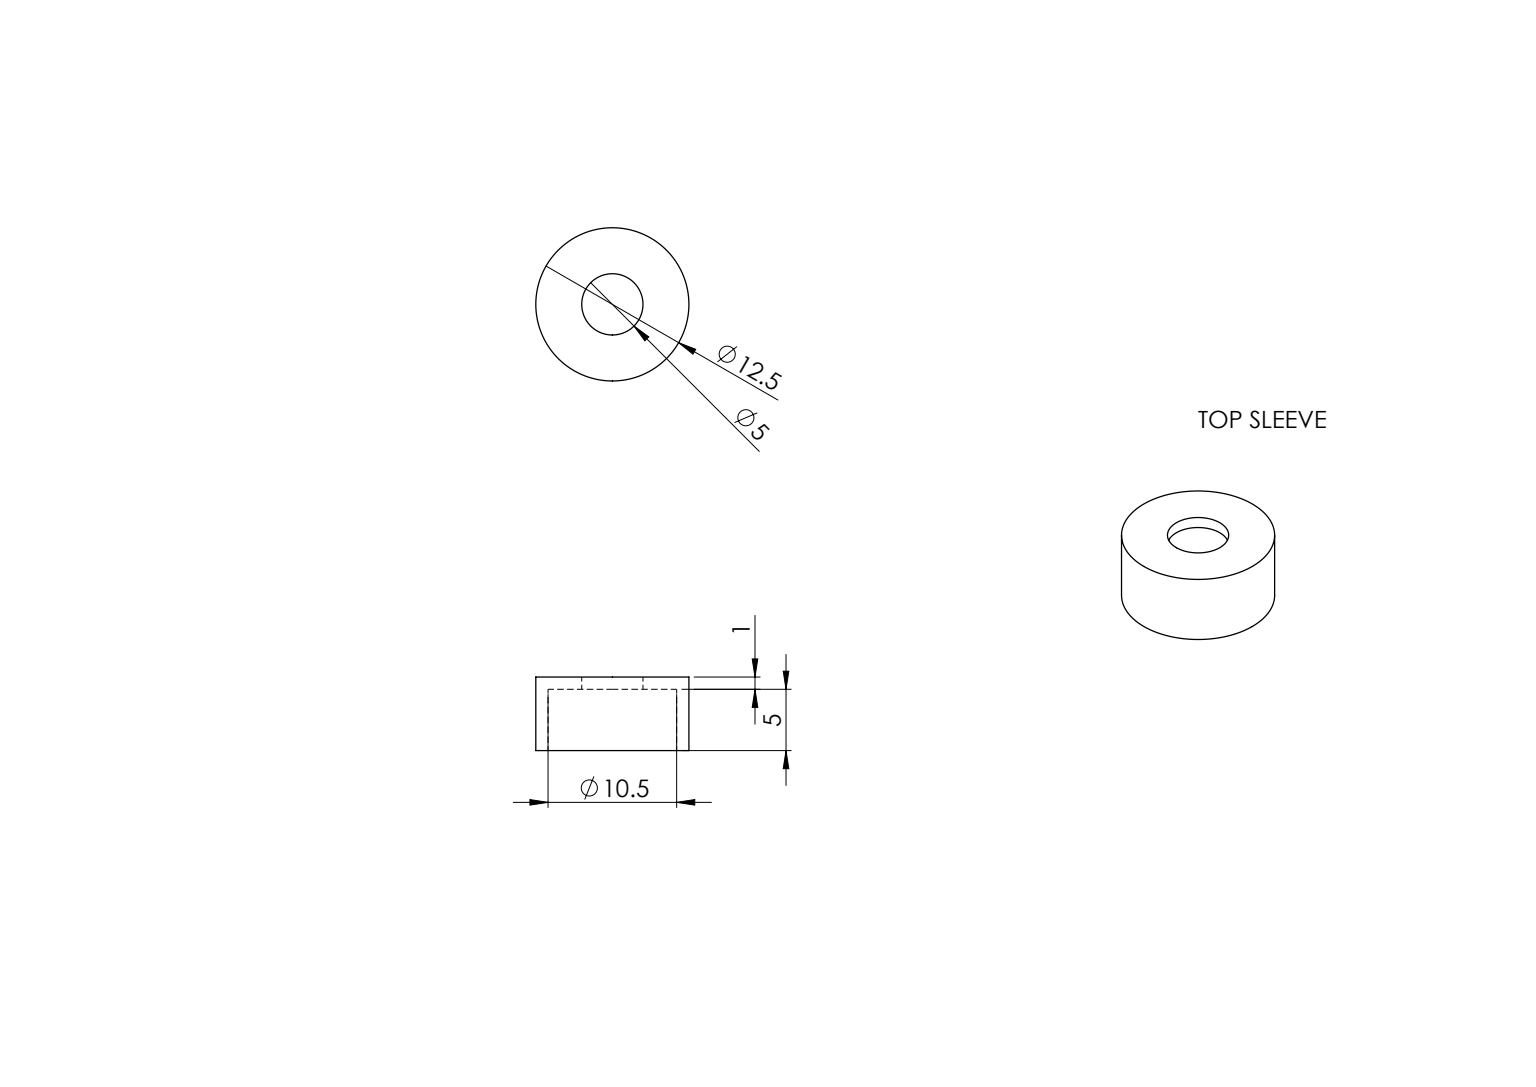
ISO-10303-21;
HEADER;
FILE_DESCRIPTION (('STEP AP214'),
    '1' );
FILE_NAME ('top sleeve.step',
    '2026-10-27T10:49:47',
    ( '' ),
    ( '' ),
    'SwSTEP 2.0',
    'SolidWorks 2026',
    '' );
FILE_SCHEMA (( 'AUTOMOTIVE_DESIGN' ));
ENDSEC;

DATA;
#1=ORIENTED_EDGE ( 'NONE', *, *, #5722, .T. ) ;
#2=FILL_AREA_STYLE ('',( #5004 ) ) ;
#66=EDGE_LOOP ( 'NONE', ( #5126, #5183, #1901, #2100 ) ) ;
#73=CYLINDRICAL_SURFACE ( 'NONE', #5825, 2.499999999999999556 ) ;
#128=DIRECTION ( 'NONE',  ( 0.000000000000000000, 0.000000000000000000, 1.000000000000000000 ) ) ;
#129=AXIS2_PLACEMENT_3D ( 'NONE', #454, #8273, #5425 ) ;
#179=VERTEX_POINT ( 'NONE', #5659 ) ;
#187=VERTEX_POINT ( 'NONE', #5479 ) ;
#213=DIRECTION ( 'NONE',  ( 0.000000000000000000, 1.000000000000000000, 0.000000000000000000 ) ) ;
#302=AXIS2_PLACEMENT_3D ( 'NONE', #4792, #7636, #6980 ) ;
#320=ORIENTED_EDGE ( 'NONE', *, *, #3522, .T. ) ;
#446=STYLED_ITEM('',(#9211),#2174);
#454=CARTESIAN_POINT ( 'NONE',  ( 0.000000000000000000, 69.99999999999998579, 0.000000000000000000 ) ) ;
#543=CARTESIAN_POINT ( 'NONE',  ( 0.000000000000000000, 69.99999999999998579, 0.000000000000000000 ) ) ;
#587=FACE_BOUND ( 'NONE', #2803, .T. ) ;
#600=AXIS2_PLACEMENT_3D ( 'NONE', #1254, #6968, #5476 ) ;
#654=( LENGTH_UNIT ( ) NAMED_UNIT ( * ) SI_UNIT ( .MILLI., .METRE. ) );
#666=CARTESIAN_POINT ( 'NONE',  ( 0.000000000000000000, 76.00000000000000000, -2.499999999999999556 ) ) ;
#689=CARTESIAN_POINT ( 'NONE',  ( 3.061616997868382648E-16, 76.00000000000000000, 2.499999999999999556 ) ) ;
#693=( NAMED_UNIT ( * ) PLANE_ANGLE_UNIT ( ) SI_UNIT ( $, .RADIAN. ) );
#736=ORIENTED_EDGE ( 'NONE', *, *, #3059, .T. ) ;
#780=AXIS2_PLACEMENT_3D ( 'NONE', #6952, #8529, #7794 ) ;
#805=DIRECTION ( 'NONE',  ( 0.000000000000000000, 1.000000000000000000, 0.000000000000000000 ) ) ;
#808=EDGE_LOOP ( 'NONE', ( #7978, #931, #7565, #1484 ) ) ;
#827=CARTESIAN_POINT ( 'NONE',  ( 0.000000000000000000, 75.00000000000000000, 0.000000000000000000 ) ) ;
#850=MECHANICAL_DESIGN_GEOMETRIC_PRESENTATION_REPRESENTATION('',(#4576),#5468);
#856=ORIENTED_EDGE ( 'NONE', *, *, #3685, .T. ) ;
#888=AXIS2_PLACEMENT_3D ( 'NONE', #4026, #9081, #6861 ) ;
#890=CIRCLE ( 'NONE', #3281, 5.250000000000000000 ) ;
#909=CARTESIAN_POINT ( 'NONE',  ( 0.000000000000000000, 75.00000000000000000, 0.000000000000000000 ) ) ;
#931=ORIENTED_EDGE ( 'NONE', *, *, #6120, .T. ) ;
#957=EDGE_CURVE ( 'NONE', #7496, #1130, #5197, .T. ) ;
#992=ORIENTED_EDGE ( 'NONE', *, *, #8749, .T. ) ;
#1009=PRODUCT_DEFINITION_FORMATION_WITH_SPECIFIED_SOURCE ( 'ANY', '', #1433, .NOT_KNOWN. ) ;
#1032=DIRECTION ( 'NONE',  ( 0.000000000000000000, 0.000000000000000000, 1.000000000000000000 ) ) ;
#1088=FACE_OUTER_BOUND ( 'NONE', #5599, .T. ) ;
#1125=EDGE_CURVE ( 'NONE', #8145, #1171, #1682, .T. ) ;
#1130=VERTEX_POINT ( 'NONE', #4733 ) ;
#1150=ORIENTED_EDGE ( 'NONE', *, *, #2707, .F. ) ;
#1166=VERTEX_POINT ( 'NONE', #3351 ) ;
#1171=VERTEX_POINT ( 'NONE', #9055 ) ;
#1199=ADVANCED_FACE ( 'NONE', ( #5698 ), #73, .F. ) ;
#1207=AXIS2_PLACEMENT_3D ( 'NONE', #827, #8513, #128 ) ;
#1232=CARTESIAN_POINT ( 'NONE',  ( 0.000000000000000000, 69.99999999999998579, 0.000000000000000000 ) ) ;
#1254=CARTESIAN_POINT ( 'NONE',  ( 0.000000000000000000, 76.00000000000000000, 0.000000000000000000 ) ) ;
#1264=FACE_OUTER_BOUND ( 'NONE', #5853, .T. ) ;
#1380=CARTESIAN_POINT ( 'NONE',  ( 0.000000000000000000, 76.00000000000000000, 0.000000000000000000 ) ) ;
#1396=SURFACE_SIDE_STYLE ('',( #4281 ) ) ;
#1433=PRODUCT ( 'top sleeve', 'top sleeve', '', ( #6229 ) ) ;
#1478=CIRCLE ( 'NONE', #6676, 5.250000000000000000 ) ;
#1484=ORIENTED_EDGE ( 'NONE', *, *, #1125, .F. ) ;
#1487=AXIS2_PLACEMENT_3D ( 'NONE', #3149, #8300, #8894 ) ;
#1496=EDGE_CURVE ( 'NONE', #1166, #179, #8185, .T. ) ;
#1537=DIRECTION ( 'NONE',  ( 0.000000000000000000, 1.000000000000000000, 0.000000000000000000 ) ) ;
#1623=ORIENTED_EDGE ( 'NONE', *, *, #8749, .F. ) ;
#1627=EDGE_LOOP ( 'NONE', ( #6721, #320, #992, #4948 ) ) ;
#1682=CIRCLE ( 'NONE', #6140, 6.250000000000000000 ) ;
#1693=CIRCLE ( 'NONE', #8384, 5.250000000000000000 ) ;
#1793=ORIENTED_EDGE ( 'NONE', *, *, #3059, .F. ) ;
#1801=DIRECTION ( 'NONE',  ( 0.000000000000000000, 1.000000000000000000, 0.000000000000000000 ) ) ;
#1804=UNCERTAINTY_MEASURE_WITH_UNIT (LENGTH_MEASURE( 1.000000000000000082E-05 ), #654, 'distance_accuracy_value', 'NONE');
#1807=VECTOR ( 'NONE', #8585, 1000.000000000000000 ) ;
#1857=AXIS2_PLACEMENT_3D ( 'NONE', #1232, #7558, #8853 ) ;
#1901=ORIENTED_EDGE ( 'NONE', *, *, #957, .T. ) ;
#1910=DIRECTION ( 'NONE',  ( -0.000000000000000000, -1.000000000000000000, -0.000000000000000000 ) ) ;
#1931=FACE_BOUND ( 'NONE', #7456, .T. ) ;
#1975=ADVANCED_FACE ( 'NONE', ( #1264, #5489 ), #4702, .T. ) ;
#1998=DIRECTION ( 'NONE',  ( 0.000000000000000000, 0.000000000000000000, 1.000000000000000000 ) ) ;
#2017=CARTESIAN_POINT ( 'NONE',  ( 0.000000000000000000, 69.99999999999998579, 6.250000000000000000 ) ) ;
#2072=EDGE_CURVE ( 'NONE', #1130, #187, #3438, .T. ) ;
#2082=DIRECTION ( 'NONE',  ( 0.000000000000000000, 0.000000000000000000, -1.000000000000000000 ) ) ;
#2100=ORIENTED_EDGE ( 'NONE', *, *, #2072, .T. ) ;
#2122=VERTEX_POINT ( 'NONE', #689 ) ;
#2143=SURFACE_STYLE_USAGE ( .BOTH. , #1396 ) ;
#2174=MANIFOLD_SOLID_BREP ( 'Boss-Extrude3', #3869 ) ;
#2188=ORIENTED_EDGE ( 'NONE', *, *, #1496, .F. ) ;
#2251=DIRECTION ( 'NONE',  ( 0.000000000000000000, 0.000000000000000000, 1.000000000000000000 ) ) ;
#2286=CIRCLE ( 'NONE', #6736, 6.250000000000000000 ) ;
#2365=EDGE_CURVE ( 'NONE', #179, #8145, #3524, .T. ) ;
#2427=APPLICATION_CONTEXT ( 'automotive_design' ) ;
#2443=DIRECTION ( 'NONE',  ( 0.000000000000000000, 1.000000000000000000, 0.000000000000000000 ) ) ;
#2453=DIRECTION ( 'NONE',  ( 0.000000000000000000, 0.000000000000000000, 1.000000000000000000 ) ) ;
#2456=UNCERTAINTY_MEASURE_WITH_UNIT (LENGTH_MEASURE( 1.000000000000000082E-05 ), #8517, 'distance_accuracy_value', 'NONE');
#2484=FACE_OUTER_BOUND ( 'NONE', #8918, .T. ) ;
#2497=FACE_OUTER_BOUND ( 'NONE', #808, .T. ) ;
#2558=CYLINDRICAL_SURFACE ( 'NONE', #129, 5.250000000000000000 ) ;
#2609=FACE_OUTER_BOUND ( 'NONE', #1627, .T. ) ;
#2652=( NAMED_UNIT ( * ) PLANE_ANGLE_UNIT ( ) SI_UNIT ( $, .RADIAN. ) );
#2690=VECTOR ( 'NONE', #7111, 1000.000000000000000 ) ;
#2699=CARTESIAN_POINT ( 'NONE',  ( 0.000000000000000000, 69.99999999999998579, 5.250000000000000000 ) ) ;
#2707=EDGE_CURVE ( 'NONE', #6263, #4547, #3442, .T. ) ;
#2726=CARTESIAN_POINT ( 'NONE',  ( 6.429395695523604153E-16, 69.99999999999998579, -5.250000000000000000 ) ) ;
#2753=APPLICATION_CONTEXT ( 'automotive_design' ) ;
#2768=ADVANCED_FACE ( 'NONE', ( #2497 ), #4083, .T. ) ;
#2803=EDGE_LOOP ( 'NONE', ( #4036, #3583 ) ) ;
#2837=CARTESIAN_POINT ( 'NONE',  ( 0.000000000000000000, 76.00000000000000000, 0.000000000000000000 ) ) ;
#2850=ADVANCED_FACE ( 'NONE', ( #587, #7088 ), #7798, .F. ) ;
#2996=AXIS2_PLACEMENT_3D ( 'NONE', #543, #1801, #6871 ) ;
#3006=DIRECTION ( 'NONE',  ( 0.000000000000000000, 1.000000000000000000, 0.000000000000000000 ) ) ;
#3059=EDGE_CURVE ( 'NONE', #2122, #4547, #4854, .T. ) ;
#3064=EDGE_CURVE ( 'NONE', #8472, #7496, #890, .T. ) ;
#3106=EDGE_CURVE ( 'NONE', #1171, #8145, #5500, .T. ) ;
#3149=CARTESIAN_POINT ( 'NONE',  ( 0.000000000000000000, 69.99999999999998579, 0.000000000000000000 ) ) ;
#3162=CARTESIAN_POINT ( 'NONE',  ( 0.000000000000000000, 69.99999999999998579, 5.250000000000000000 ) ) ;
#3210=DIRECTION ( 'NONE',  ( 0.000000000000000000, 1.000000000000000000, 0.000000000000000000 ) ) ;
#3227=EDGE_CURVE ( 'NONE', #4547, #6263, #5645, .T. ) ;
#3277=DIRECTION ( 'NONE',  ( 0.000000000000000000, -0.000000000000000000, 1.000000000000000000 ) ) ;
#3281=AXIS2_PLACEMENT_3D ( 'NONE', #7929, #3006, #7182 ) ;
#3320=CIRCLE ( 'NONE', #780, 2.499999999999999556 ) ;
#3351=CARTESIAN_POINT ( 'NONE',  ( 0.000000000000000000, 69.99999999999998579, 6.250000000000000000 ) ) ;
#3396=CARTESIAN_POINT ( 'NONE',  ( 0.000000000000000000, 76.00000000000000000, 0.000000000000000000 ) ) ;
#3438=CIRCLE ( 'NONE', #1207, 5.250000000000000000 ) ;
#3442=CIRCLE ( 'NONE', #8629, 2.499999999999999556 ) ;
#3522=EDGE_CURVE ( 'NONE', #8472, #187, #4278, .T. ) ;
#3524=LINE ( 'NONE', #9099, #1807 ) ;
#3583=ORIENTED_EDGE ( 'NONE', *, *, #3227, .T. ) ;
#3673=SHAPE_REPRESENTATION_RELATIONSHIP ( 'NONE' , 'NONE' ,  #3797, #7073 ) ;
#3685=EDGE_CURVE ( 'NONE', #2122, #4375, #8478, .T. ) ;
#3784=ADVANCED_FACE ( 'NONE', ( #6485 ), #7849, .F. ) ;
#3797=SHAPE_REPRESENTATION ( 'top sleeve', ( #888 ), #6054 ) ;
#3869=CLOSED_SHELL ( 'NONE', ( #1199, #7781, #4657, #2768, #5305, #6558, #2850, #1975, #3784 ) ) ;
#3883=DIRECTION ( 'NONE',  ( 0.000000000000000000, 0.000000000000000000, 1.000000000000000000 ) ) ;
#3888=( GEOMETRIC_REPRESENTATION_CONTEXT ( 3 ) GLOBAL_UNCERTAINTY_ASSIGNED_CONTEXT ( ( #4539 ) ) GLOBAL_UNIT_ASSIGNED_CONTEXT ( ( #4046, #2652, #5427 ) ) REPRESENTATION_CONTEXT ( 'NONE', 'WORKASPACE' ) );
#3945=PRODUCT_DEFINITION_CONTEXT ( 'detailed design', #2427, 'design' ) ;
#3974=CARTESIAN_POINT ( 'NONE',  ( 3.061616997868382648E-16, 75.00000000000000000, 2.499999999999999556 ) ) ;
#4026=CARTESIAN_POINT ( 'NONE',  ( 0.000000000000000000, 0.000000000000000000, 0.000000000000000000 ) ) ;
#4036=ORIENTED_EDGE ( 'NONE', *, *, #2707, .T. ) ;
#4046=( LENGTH_UNIT ( ) NAMED_UNIT ( * ) SI_UNIT ( .MILLI., .METRE. ) );
#4060=EDGE_LOOP ( 'NONE', ( #5251, #7001 ) ) ;
#4067=PLANE ( 'NONE',  #8072 ) ;
#4083=CYLINDRICAL_SURFACE ( 'NONE', #2996, 6.250000000000000000 ) ;
#4093=LINE ( 'NONE', #5289, #8080 ) ;
#4105=ORIENTED_EDGE ( 'NONE', *, *, #3064, .T. ) ;
#4169=AXIS2_PLACEMENT_3D ( 'NONE', #8065, #2443, #8256 ) ;
#4214=DIRECTION ( 'NONE',  ( 0.000000000000000000, -0.000000000000000000, 1.000000000000000000 ) ) ;
#4225=DIRECTION ( 'NONE',  ( 0.000000000000000000, 0.000000000000000000, -1.000000000000000000 ) ) ;
#4278=LINE ( 'NONE', #7246, #2690 ) ;
#4281=SURFACE_STYLE_FILL_AREA ( #2 ) ;
#4302=EDGE_CURVE ( 'NONE', #4375, #2122, #3320, .T. ) ;
#4325=ORIENTED_EDGE ( 'NONE', *, *, #3227, .F. ) ;
#4375=VERTEX_POINT ( 'NONE', #666 ) ;
#4380=DIRECTION ( 'NONE',  ( 0.000000000000000000, 0.000000000000000000, 1.000000000000000000 ) ) ;
#4387=CARTESIAN_POINT ( 'NONE',  ( 0.000000000000000000, 75.00000000000000000, 0.000000000000000000 ) ) ;
#4393=DIRECTION ( 'NONE',  ( -0.000000000000000000, -1.000000000000000000, -0.000000000000000000 ) ) ;
#4459=VECTOR ( 'NONE', #4393, 1000.000000000000000 ) ;
#4539=UNCERTAINTY_MEASURE_WITH_UNIT (LENGTH_MEASURE( 1.000000000000000082E-05 ), #4046, 'distance_accuracy_value', 'NONE');
#4547=VERTEX_POINT ( 'NONE', #3974 ) ;
#4548=CARTESIAN_POINT ( 'NONE',  ( 0.000000000000000000, 69.99999999999998579, 0.000000000000000000 ) ) ;
#4576=STYLED_ITEM ( 'NONE', ( #4964 ), #7073 ) ;
#4621=CARTESIAN_POINT ( 'NONE',  ( 0.000000000000000000, 69.99999999999998579, 0.000000000000000000 ) ) ;
#4657=ADVANCED_FACE ( 'NONE', ( #2484 ), #6104, .T. ) ;
#4693=SHAPE_DEFINITION_REPRESENTATION ( #7231, #3797 ) ;
#4702=PLANE ( 'NONE',  #302 ) ;
#4733=CARTESIAN_POINT ( 'NONE',  ( 0.000000000000000000, 75.00000000000000000, 5.250000000000000000 ) ) ;
#4759=DIRECTION ( 'NONE',  ( 0.000000000000000000, 1.000000000000000000, 0.000000000000000000 ) ) ;
#4792=CARTESIAN_POINT ( 'NONE',  ( 0.000000000000000000, 76.00000000000000000, 0.000000000000000000 ) ) ;
#4802=CARTESIAN_POINT ( 'NONE',  ( 0.000000000000000000, 69.99999999999998579, 0.000000000000000000 ) ) ;
#4854=LINE ( 'NONE', #7700, #4459 ) ;
#4948=ORIENTED_EDGE ( 'NONE', *, *, #957, .F. ) ;
#4964=PRESENTATION_STYLE_ASSIGNMENT (( #2143 ) ) ;
#4981=DIRECTION ( 'NONE',  ( 0.000000000000000000, 1.000000000000000000, 0.000000000000000000 ) ) ;
#5004=FILL_AREA_STYLE_COLOUR ( '', #7846 ) ;
#5075=CARTESIAN_POINT ( 'NONE',  ( 0.000000000000000000, 76.00000000000000000, 0.000000000000000000 ) ) ;
#5126=ORIENTED_EDGE ( 'NONE', *, *, #3522, .F. ) ;
#5183=ORIENTED_EDGE ( 'NONE', *, *, #5647, .F. ) ;
#5197=LINE ( 'NONE', #2699, #7034 ) ;
#5230=ORIENTED_EDGE ( 'NONE', *, *, #1496, .T. ) ;
#5237=DIRECTION ( 'NONE',  ( 0.000000000000000000, 1.000000000000000000, 0.000000000000000000 ) ) ;
#5251=ORIENTED_EDGE ( 'NONE', *, *, #4302, .F. ) ;
#5254=EDGE_LOOP ( 'NONE', ( #1793, #856, #1, #4325 ) ) ;
#5260=EDGE_CURVE ( 'NONE', #1166, #1171, #6055, .T. ) ;
#5289=CARTESIAN_POINT ( 'NONE',  ( 0.000000000000000000, 76.00000000000000000, -2.499999999999999556 ) ) ;
#5305=ADVANCED_FACE ( 'NONE', ( #1931, #1088 ), #4067, .F. ) ;
#5338=MECHANICAL_DESIGN_GEOMETRIC_PRESENTATION_REPRESENTATION('',(#446),#3888);
#5391=ORIENTED_EDGE ( 'NONE', *, *, #2072, .F. ) ;
#5425=DIRECTION ( 'NONE',  ( 0.000000000000000000, 0.000000000000000000, 1.000000000000000000 ) ) ;
#5427=( NAMED_UNIT ( * ) SI_UNIT ( $, .STERADIAN. ) SOLID_ANGLE_UNIT ( ) );
#5468=( GEOMETRIC_REPRESENTATION_CONTEXT ( 3 ) GLOBAL_UNCERTAINTY_ASSIGNED_CONTEXT ( ( #1804 ) ) GLOBAL_UNIT_ASSIGNED_CONTEXT ( ( #654, #7861, #6319 ) ) REPRESENTATION_CONTEXT ( 'NONE', 'WORKASPACE' ) );
#5475=DIRECTION ( 'NONE',  ( 0.000000000000000000, 1.000000000000000000, 0.000000000000000000 ) ) ;
#5476=DIRECTION ( 'NONE',  ( 0.000000000000000000, 0.000000000000000000, 1.000000000000000000 ) ) ;
#5479=CARTESIAN_POINT ( 'NONE',  ( 6.429395695523604153E-16, 75.00000000000000000, -5.250000000000000000 ) ) ;
#5489=FACE_BOUND ( 'NONE', #4060, .T. ) ;
#5500=CIRCLE ( 'NONE', #7734, 6.250000000000000000 ) ;
#5599=EDGE_LOOP ( 'NONE', ( #2188, #8815 ) ) ;
#5645=CIRCLE ( 'NONE', #4169, 2.499999999999999556 ) ;
#5647=EDGE_CURVE ( 'NONE', #7496, #8472, #1693, .T. ) ;
#5659=CARTESIAN_POINT ( 'NONE',  ( 7.654042494670957606E-16, 69.99999999999998579, -6.250000000000000000 ) ) ;
#5698=FACE_OUTER_BOUND ( 'NONE', #7995, .T. ) ;
#5722=EDGE_CURVE ( 'NONE', #4375, #6263, #4093, .T. ) ;
#5816=CARTESIAN_POINT ( 'NONE',  ( 0.000000000000000000, 69.99999999999998579, 0.000000000000000000 ) ) ;
#5825=AXIS2_PLACEMENT_3D ( 'NONE', #1380, #8457, #2082 ) ;
#5853=EDGE_LOOP ( 'NONE', ( #7431, #8166 ) ) ;
#5995=ORIENTED_EDGE ( 'NONE', *, *, #5260, .F. ) ;
#6054=( GEOMETRIC_REPRESENTATION_CONTEXT ( 3 ) GLOBAL_UNCERTAINTY_ASSIGNED_CONTEXT ( ( #2456 ) ) GLOBAL_UNIT_ASSIGNED_CONTEXT ( ( #8517, #693, #7025 ) ) REPRESENTATION_CONTEXT ( 'NONE', 'WORKASPACE' ) );
#6055=LINE ( 'NONE', #2017, #6727 ) ;
#6071=ORIENTED_EDGE ( 'NONE', *, *, #3106, .F. ) ;
#6104=CYLINDRICAL_SURFACE ( 'NONE', #8805, 6.250000000000000000 ) ;
#6120=EDGE_CURVE ( 'NONE', #179, #1166, #2286, .T. ) ;
#6140=AXIS2_PLACEMENT_3D ( 'NONE', #3396, #3210, #1998 ) ;
#6229=PRODUCT_CONTEXT ( 'NONE', #2753, 'mechanical' ) ;
#6263=VERTEX_POINT ( 'NONE', #6388 ) ;
#6319=( NAMED_UNIT ( * ) SI_UNIT ( $, .STERADIAN. ) SOLID_ANGLE_UNIT ( ) );
#6386=ORIENTED_EDGE ( 'NONE', *, *, #5647, .T. ) ;
#6388=CARTESIAN_POINT ( 'NONE',  ( 0.000000000000000000, 75.00000000000000000, -2.499999999999999556 ) ) ;
#6485=FACE_OUTER_BOUND ( 'NONE', #5254, .T. ) ;
#6558=ADVANCED_FACE ( 'NONE', ( #6812 ), #8942, .F. ) ;
#6660=ORIENTED_EDGE ( 'NONE', *, *, #2365, .T. ) ;
#6676=AXIS2_PLACEMENT_3D ( 'NONE', #4387, #7409, #1032 ) ;
#6721=ORIENTED_EDGE ( 'NONE', *, *, #3064, .F. ) ;
#6727=VECTOR ( 'NONE', #6943, 1000.000000000000000 ) ;
#6736=AXIS2_PLACEMENT_3D ( 'NONE', #4548, #5237, #7196 ) ;
#6812=FACE_OUTER_BOUND ( 'NONE', #66, .T. ) ;
#6861=DIRECTION ( 'NONE',  ( 1.000000000000000000, 0.000000000000000000, 0.000000000000000000 ) ) ;
#6871=DIRECTION ( 'NONE',  ( 0.000000000000000000, 0.000000000000000000, 1.000000000000000000 ) ) ;
#6943=DIRECTION ( 'NONE',  ( 0.000000000000000000, 1.000000000000000000, 0.000000000000000000 ) ) ;
#6952=CARTESIAN_POINT ( 'NONE',  ( 0.000000000000000000, 76.00000000000000000, 0.000000000000000000 ) ) ;
#6968=DIRECTION ( 'NONE',  ( 0.000000000000000000, 1.000000000000000000, 0.000000000000000000 ) ) ;
#6980=DIRECTION ( 'NONE',  ( 0.000000000000000000, -0.000000000000000000, 1.000000000000000000 ) ) ;
#7001=ORIENTED_EDGE ( 'NONE', *, *, #3685, .F. ) ;
#7025=( NAMED_UNIT ( * ) SI_UNIT ( $, .STERADIAN. ) SOLID_ANGLE_UNIT ( ) );
#7034=VECTOR ( 'NONE', #5475, 1000.000000000000000 ) ;
#7073=ADVANCED_BREP_SHAPE_REPRESENTATION ( '', ( #2174, #888 ), #6054 ) ;
#7088=FACE_OUTER_BOUND ( 'NONE', #7539, .T. ) ;
#7111=DIRECTION ( 'NONE',  ( 0.000000000000000000, 1.000000000000000000, 0.000000000000000000 ) ) ;
#7182=DIRECTION ( 'NONE',  ( 0.000000000000000000, 0.000000000000000000, 1.000000000000000000 ) ) ;
#7196=DIRECTION ( 'NONE',  ( 1.000000000000000000, 0.000000000000000000, 0.000000000000000000 ) ) ;
#7224=ORIENTED_EDGE ( 'NONE', *, *, #4302, .T. ) ;
#7229=CARTESIAN_POINT ( 'NONE',  ( 7.654042494670957606E-16, 76.00000000000000000, -6.250000000000000000 ) ) ;
#7231=PRODUCT_DEFINITION_SHAPE ( 'NONE', 'NONE',  #8320 ) ;
#7246=CARTESIAN_POINT ( 'NONE',  ( 6.429395695523604153E-16, 69.99999999999998579, -5.250000000000000000 ) ) ;
#7409=DIRECTION ( 'NONE',  ( 0.000000000000000000, 1.000000000000000000, 0.000000000000000000 ) ) ;
#7431=ORIENTED_EDGE ( 'NONE', *, *, #3106, .T. ) ;
#7435=AXIS2_PLACEMENT_3D ( 'NONE', #2837, #7713, #4225 ) ;
#7456=EDGE_LOOP ( 'NONE', ( #6386, #4105 ) ) ;
#7496=VERTEX_POINT ( 'NONE', #3162 ) ;
#7539=EDGE_LOOP ( 'NONE', ( #5391, #1623 ) ) ;
#7558=DIRECTION ( 'NONE',  ( 0.000000000000000000, 1.000000000000000000, 0.000000000000000000 ) ) ;
#7565=ORIENTED_EDGE ( 'NONE', *, *, #5260, .T. ) ;
#7636=DIRECTION ( 'NONE',  ( 0.000000000000000000, 1.000000000000000000, 0.000000000000000000 ) ) ;
#7700=CARTESIAN_POINT ( 'NONE',  ( 3.061616997868382648E-16, 76.00000000000000000, 2.499999999999999556 ) ) ;
#7713=DIRECTION ( 'NONE',  ( -0.000000000000000000, -1.000000000000000000, -0.000000000000000000 ) ) ;
#7734=AXIS2_PLACEMENT_3D ( 'NONE', #5075, #805, #2251 ) ;
#7781=ADVANCED_FACE ( 'NONE', ( #2609 ), #2558, .F. ) ;
#7794=DIRECTION ( 'NONE',  ( 0.000000000000000000, 0.000000000000000000, 1.000000000000000000 ) ) ;
#7798=PLANE ( 'NONE',  #8019 ) ;
#7846=COLOUR_RGB ( '',0.8941176470588234615, 0.8941176470588234615, 0.8941176470588234615 ) ;
#7849=CYLINDRICAL_SURFACE ( 'NONE', #7435, 2.499999999999999556 ) ;
#7861=( NAMED_UNIT ( * ) PLANE_ANGLE_UNIT ( ) SI_UNIT ( $, .RADIAN. ) );
#7929=CARTESIAN_POINT ( 'NONE',  ( 0.000000000000000000, 69.99999999999998579, 0.000000000000000000 ) ) ;
#7978=ORIENTED_EDGE ( 'NONE', *, *, #2365, .F. ) ;
#7995=EDGE_LOOP ( 'NONE', ( #7224, #736, #1150, #8618 ) ) ;
#8019=AXIS2_PLACEMENT_3D ( 'NONE', #8494, #4981, #4214 ) ;
#8065=CARTESIAN_POINT ( 'NONE',  ( 0.000000000000000000, 75.00000000000000000, 0.000000000000000000 ) ) ;
#8072=AXIS2_PLACEMENT_3D ( 'NONE', #4802, #4759, #3277 ) ;
#8080=VECTOR ( 'NONE', #1910, 1000.000000000000000 ) ;
#8145=VERTEX_POINT ( 'NONE', #7229 ) ;
#8166=ORIENTED_EDGE ( 'NONE', *, *, #1125, .T. ) ;
#8185=CIRCLE ( 'NONE', #1487, 6.250000000000000000 ) ;
#8256=DIRECTION ( 'NONE',  ( 0.000000000000000000, 0.000000000000000000, 1.000000000000000000 ) ) ;
#8273=DIRECTION ( 'NONE',  ( 0.000000000000000000, 1.000000000000000000, 0.000000000000000000 ) ) ;
#8300=DIRECTION ( 'NONE',  ( 0.000000000000000000, 1.000000000000000000, 0.000000000000000000 ) ) ;
#8320=PRODUCT_DEFINITION ( 'UNKNOWN', '', #1009, #3945 ) ;
#8384=AXIS2_PLACEMENT_3D ( 'NONE', #5816, #1537, #4380 ) ;
#8457=DIRECTION ( 'NONE',  ( -0.000000000000000000, -1.000000000000000000, -0.000000000000000000 ) ) ;
#8472=VERTEX_POINT ( 'NONE', #2726 ) ;
#8478=CIRCLE ( 'NONE', #600, 2.499999999999999556 ) ;
#8494=CARTESIAN_POINT ( 'NONE',  ( 0.000000000000000000, 75.00000000000000000, 0.000000000000000000 ) ) ;
#8513=DIRECTION ( 'NONE',  ( 0.000000000000000000, 1.000000000000000000, 0.000000000000000000 ) ) ;
#8517=( LENGTH_UNIT ( ) NAMED_UNIT ( * ) SI_UNIT ( .MILLI., .METRE. ) );
#8529=DIRECTION ( 'NONE',  ( 0.000000000000000000, 1.000000000000000000, 0.000000000000000000 ) ) ;
#8585=DIRECTION ( 'NONE',  ( 0.000000000000000000, 1.000000000000000000, 0.000000000000000000 ) ) ;
#8618=ORIENTED_EDGE ( 'NONE', *, *, #5722, .F. ) ;
#8629=AXIS2_PLACEMENT_3D ( 'NONE', #909, #213, #2453 ) ;
#8749=EDGE_CURVE ( 'NONE', #187, #1130, #1478, .T. ) ;
#8805=AXIS2_PLACEMENT_3D ( 'NONE', #4621, #8890, #3883 ) ;
#8815=ORIENTED_EDGE ( 'NONE', *, *, #6120, .F. ) ;
#8853=DIRECTION ( 'NONE',  ( 0.000000000000000000, 0.000000000000000000, 1.000000000000000000 ) ) ;
#8890=DIRECTION ( 'NONE',  ( 0.000000000000000000, 1.000000000000000000, 0.000000000000000000 ) ) ;
#8894=DIRECTION ( 'NONE',  ( 1.000000000000000000, 0.000000000000000000, 0.000000000000000000 ) ) ;
#8918=EDGE_LOOP ( 'NONE', ( #5230, #6660, #6071, #5995 ) ) ;
#8942=CYLINDRICAL_SURFACE ( 'NONE', #1857, 5.250000000000000000 ) ;
#9055=CARTESIAN_POINT ( 'NONE',  ( 0.000000000000000000, 76.00000000000000000, 6.250000000000000000 ) ) ;
#9081=DIRECTION ( 'NONE',  ( 0.000000000000000000, 0.000000000000000000, 1.000000000000000000 ) ) ;
#9099=CARTESIAN_POINT ( 'NONE',  ( 7.654042494670957606E-16, 69.99999999999998579, -6.250000000000000000 ) ) ;
#9205=COLOUR_RGB('Light Blue',0.38,0.62,0.78);
#9206=FILL_AREA_STYLE_COLOUR('',#9205);
#9207=FILL_AREA_STYLE('',(#9206));
#9208=SURFACE_STYLE_FILL_AREA(#9207);
#9209=SURFACE_SIDE_STYLE('',(#9208));
#9210=SURFACE_STYLE_USAGE(.BOTH.,#9209);
#9211=PRESENTATION_STYLE_ASSIGNMENT((#9210));
ENDSEC;
END-ISO-10303-21;
